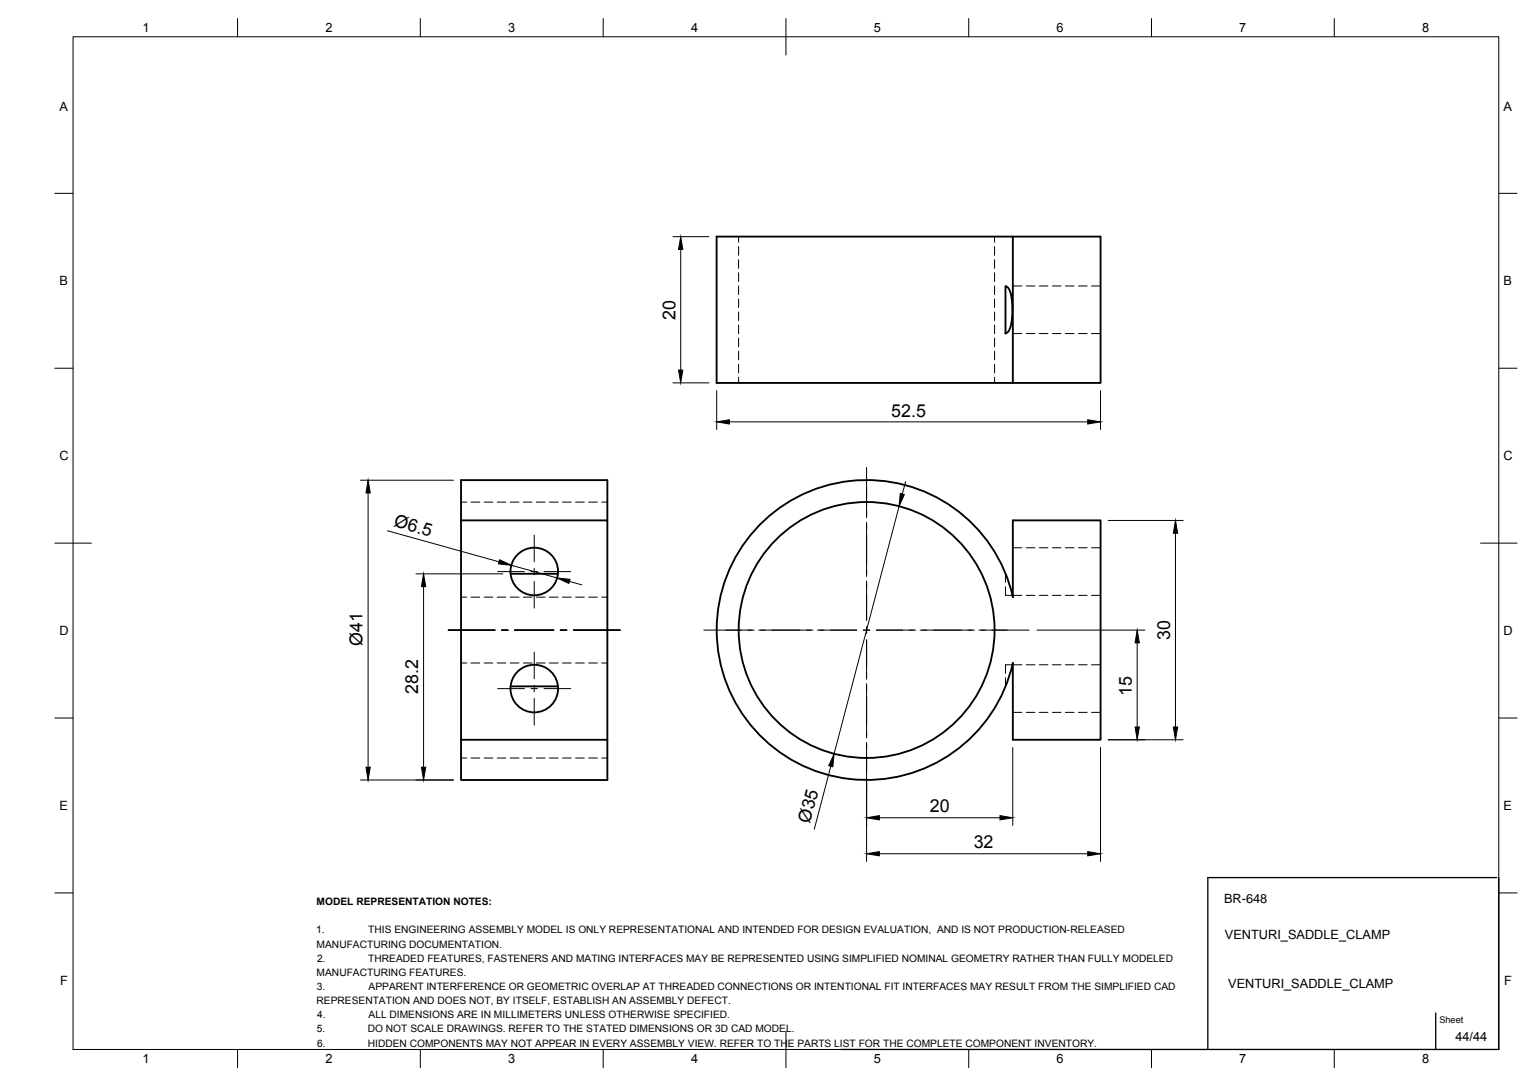
ISO-10303-21;
HEADER;
FILE_DESCRIPTION((''),'2;1');
FILE_NAME('VENTURI_SADDLE_CLAMP.step','2026-10-01T22:05:39-07:00',(''),(''),'','','');
FILE_SCHEMA (('AUTOMOTIVE_DESIGN { 1 0 10303 214 3 1 1 }'));
ENDSEC;
DATA;
#10=MECHANICAL_DESIGN_GEOMETRIC_PRESENTATION_REPRESENTATION('',(#640),#24628);
#556=SHAPE_REPRESENTATION_RELATIONSHIP('SRR','None',#24830,#598) ;
#598=ADVANCED_BREP_SHAPE_REPRESENTATION('',(#679),#24620) ;
#640=STYLED_ITEM('',(#25037),#679) ;
#679=MANIFOLD_SOLID_BREP('VENTURI_SADDLE_CLAMP',#13182) ;
#934=FACE_BOUND('',#4679,.T.) ;
#935=FACE_BOUND('',#4681,.T.) ;
#936=FACE_BOUND('',#4683,.T.) ;
#937=FACE_BOUND('',#4684,.T.) ;
#938=FACE_BOUND('',#4688,.T.) ;
#939=FACE_BOUND('',#4690,.T.) ;
#940=FACE_BOUND('',#4691,.T.) ;
#941=FACE_BOUND('',#4694,.T.) ;
#999=B_SPLINE_CURVE_WITH_KNOTS('',3,(#24196,#24197,#24198,#24199,#24200,
#24201,#24202,#24203,#24204,#24205,#24206,#24207,#24208,#24209,#24210,#24211,
#24212,#24213,#24214),.UNSPECIFIED.,.F.,.F.,(4,2,2,2,3,2,2,2,4),(-0.471793481292107,
-0.373843585675949,-0.243618913657373,-0.121809456828687,0.,0.121809456828687,
0.243618913657373,0.373843585675949,0.471793481292107),.UNSPECIFIED.) ;
#1000=B_SPLINE_CURVE_WITH_KNOTS('',3,(#24227,#24228,#24229,#24230,#24231,
#24232,#24233,#24234,#24235,#24236,#24237,#24238,#24239,#24240,#24241,#24242,
#24243,#24244),.UNSPECIFIED.,.F.,.F.,(4,2,2,2,2,2,2,2,4),(0.554019722357309,
0.651969617973467,0.782194289992043,0.904003746820729,1.02581320364942,
1.1476226604781,1.26943211730679,1.39965678932537,1.49760668494152),
 .UNSPECIFIED.) ;
#1736=LINE('',#24187,#2572) ;
#1737=LINE('',#24193,#2573) ;
#1738=LINE('',#24218,#2574) ;
#1739=LINE('',#24224,#2575) ;
#1740=LINE('',#24248,#2576) ;
#1741=LINE('',#24250,#2577) ;
#1742=LINE('',#24252,#2578) ;
#1743=LINE('',#24253,#2579) ;
#1744=LINE('',#24257,#2580) ;
#1745=LINE('',#24259,#2581) ;
#1746=LINE('',#24261,#2582) ;
#1747=LINE('',#24262,#2583) ;
#1748=LINE('',#24266,#2584) ;
#1749=LINE('',#24268,#2585) ;
#1750=LINE('',#24270,#2586) ;
#1751=LINE('',#24271,#2587) ;
#1752=LINE('',#24273,#2588) ;
#1753=LINE('',#24274,#2589) ;
#1754=LINE('',#24276,#2590) ;
#1755=LINE('',#24277,#2591) ;
#1756=LINE('',#24286,#2592) ;
#2572=VECTOR('',#19353,1.) ;
#2573=VECTOR('',#19360,0.325) ;
#2574=VECTOR('',#19367,1.) ;
#2575=VECTOR('',#19374,0.325) ;
#2576=VECTOR('',#19381,1.) ;
#2577=VECTOR('',#19382,1.) ;
#2578=VECTOR('',#19383,1.) ;
#2579=VECTOR('',#19384,1.) ;
#2580=VECTOR('',#19387,1.) ;
#2581=VECTOR('',#19388,1.) ;
#2582=VECTOR('',#19389,1.) ;
#2583=VECTOR('',#19390,1.) ;
#2584=VECTOR('',#19393,1.) ;
#2585=VECTOR('',#19394,1.) ;
#2586=VECTOR('',#19395,1.) ;
#2587=VECTOR('',#19396,1.) ;
#2588=VECTOR('',#19399,1.) ;
#2589=VECTOR('',#19400,1.) ;
#2590=VECTOR('',#19403,1.) ;
#2591=VECTOR('',#19404,1.) ;
#2592=VECTOR('',#19417,1.75) ;
#2938=CYLINDRICAL_SURFACE('',#15267,0.325) ;
#2939=CYLINDRICAL_SURFACE('',#15270,0.325) ;
#2940=CYLINDRICAL_SURFACE('',#15273,0.325) ;
#2941=CYLINDRICAL_SURFACE('',#15276,0.325) ;
#2942=CYLINDRICAL_SURFACE('',#15285,2.05) ;
#2943=CYLINDRICAL_SURFACE('',#15287,1.75) ;
#3657=FACE_OUTER_BOUND('',#4672,.T.) ;
#3658=FACE_OUTER_BOUND('',#4673,.T.) ;
#3659=FACE_OUTER_BOUND('',#4674,.T.) ;
#3660=FACE_OUTER_BOUND('',#4675,.T.) ;
#3661=FACE_OUTER_BOUND('',#4676,.T.) ;
#3662=FACE_OUTER_BOUND('',#4677,.T.) ;
#3663=FACE_OUTER_BOUND('',#4678,.T.) ;
#3664=FACE_OUTER_BOUND('',#4680,.T.) ;
#3665=FACE_OUTER_BOUND('',#4682,.T.) ;
#3666=FACE_OUTER_BOUND('',#4685,.T.) ;
#3667=FACE_OUTER_BOUND('',#4686,.T.) ;
#3668=FACE_OUTER_BOUND('',#4687,.T.) ;
#3669=FACE_OUTER_BOUND('',#4689,.T.) ;
#3670=FACE_OUTER_BOUND('',#4692,.T.) ;
#3671=FACE_OUTER_BOUND('',#4693,.T.) ;
#4672=EDGE_LOOP('',(#11737,#11738)) ;
#4673=EDGE_LOOP('',(#11739,#11740,#11741,#11742)) ;
#4674=EDGE_LOOP('',(#11743,#11744)) ;
#4675=EDGE_LOOP('',(#11745,#11746)) ;
#4676=EDGE_LOOP('',(#11747,#11748,#11749,#11750)) ;
#4677=EDGE_LOOP('',(#11751,#11752)) ;
#4678=EDGE_LOOP('',(#11753,#11754,#11755,#11756)) ;
#4679=EDGE_LOOP('',(#11757)) ;
#4680=EDGE_LOOP('',(#11758,#11759,#11760,#11761)) ;
#4681=EDGE_LOOP('',(#11762)) ;
#4682=EDGE_LOOP('',(#11763,#11764,#11765,#11766)) ;
#4683=EDGE_LOOP('',(#11767)) ;
#4684=EDGE_LOOP('',(#11768)) ;
#4685=EDGE_LOOP('',(#11769,#11770,#11771,#11772)) ;
#4686=EDGE_LOOP('',(#11773,#11774,#11775,#11776)) ;
#4687=EDGE_LOOP('',(#11777,#11778,#11779,#11780,#11781,#11782)) ;
#4688=EDGE_LOOP('',(#11783)) ;
#4689=EDGE_LOOP('',(#11784,#11785,#11786,#11787)) ;
#4690=EDGE_LOOP('',(#11788,#11789)) ;
#4691=EDGE_LOOP('',(#11790,#11791)) ;
#4692=EDGE_LOOP('',(#11792,#11793,#11794,#11795)) ;
#4693=EDGE_LOOP('',(#11796,#11797,#11798,#11799,#11800,#11801)) ;
#4694=EDGE_LOOP('',(#11802)) ;
#5511=CIRCLE('',#15266,0.325) ;
#5512=CIRCLE('',#15268,0.325) ;
#5513=CIRCLE('',#15269,0.325) ;
#5514=CIRCLE('',#15272,0.325) ;
#5515=CIRCLE('',#15274,0.325) ;
#5516=CIRCLE('',#15275,0.325) ;
#5517=CIRCLE('',#15283,2.05) ;
#5518=CIRCLE('',#15284,1.75) ;
#5519=CIRCLE('',#15286,2.05) ;
#5520=CIRCLE('',#15288,1.75) ;
#6647=VERTEX_POINT('',#24185) ;
#6648=VERTEX_POINT('',#24186) ;
#6649=VERTEX_POINT('',#24190) ;
#6650=VERTEX_POINT('',#24192) ;
#6651=VERTEX_POINT('',#24216) ;
#6652=VERTEX_POINT('',#24217) ;
#6653=VERTEX_POINT('',#24221) ;
#6654=VERTEX_POINT('',#24223) ;
#6655=VERTEX_POINT('',#24246) ;
#6656=VERTEX_POINT('',#24247) ;
#6657=VERTEX_POINT('',#24249) ;
#6658=VERTEX_POINT('',#24251) ;
#6659=VERTEX_POINT('',#24255) ;
#6660=VERTEX_POINT('',#24256) ;
#6661=VERTEX_POINT('',#24258) ;
#6662=VERTEX_POINT('',#24260) ;
#6663=VERTEX_POINT('',#24264) ;
#6664=VERTEX_POINT('',#24265) ;
#6665=VERTEX_POINT('',#24267) ;
#6666=VERTEX_POINT('',#24269) ;
#6667=VERTEX_POINT('',#24280) ;
#6668=VERTEX_POINT('',#24285) ;
#8358=EDGE_CURVE('',#6647,#6648,#1736,.T.) ;
#8359=EDGE_CURVE('',#6648,#6647,#5511,.T.) ;
#8360=EDGE_CURVE('',#6649,#6649,#5512,.T.) ;
#8361=EDGE_CURVE('',#6649,#6650,#1737,.T.) ;
#8362=EDGE_CURVE('',#6650,#6650,#5513,.T.) ;
#8363=EDGE_CURVE('',#6648,#6647,#999,.T.) ;
#8364=EDGE_CURVE('',#6651,#6652,#1738,.T.) ;
#8365=EDGE_CURVE('',#6652,#6651,#5514,.T.) ;
#8366=EDGE_CURVE('',#6653,#6653,#5515,.T.) ;
#8367=EDGE_CURVE('',#6653,#6654,#1739,.T.) ;
#8368=EDGE_CURVE('',#6654,#6654,#5516,.T.) ;
#8369=EDGE_CURVE('',#6652,#6651,#1000,.T.) ;
#8370=EDGE_CURVE('',#6655,#6656,#1740,.T.) ;
#8371=EDGE_CURVE('',#6655,#6657,#1741,.T.) ;
#8372=EDGE_CURVE('',#6657,#6658,#1742,.T.) ;
#8373=EDGE_CURVE('',#6658,#6656,#1743,.T.) ;
#8374=EDGE_CURVE('',#6659,#6660,#1744,.T.) ;
#8375=EDGE_CURVE('',#6659,#6661,#1745,.T.) ;
#8376=EDGE_CURVE('',#6661,#6662,#1746,.T.) ;
#8377=EDGE_CURVE('',#6662,#6660,#1747,.T.) ;
#8378=EDGE_CURVE('',#6663,#6664,#1748,.T.) ;
#8379=EDGE_CURVE('',#6664,#6665,#1749,.T.) ;
#8380=EDGE_CURVE('',#6665,#6666,#1750,.T.) ;
#8381=EDGE_CURVE('',#6666,#6663,#1751,.T.) ;
#8382=EDGE_CURVE('',#6657,#6665,#1752,.T.) ;
#8383=EDGE_CURVE('',#6658,#6664,#1753,.T.) ;
#8384=EDGE_CURVE('',#6661,#6663,#1754,.T.) ;
#8385=EDGE_CURVE('',#6662,#6666,#1755,.T.) ;
#8386=EDGE_CURVE('',#6655,#6660,#5517,.T.) ;
#8387=EDGE_CURVE('',#6667,#6667,#5518,.T.) ;
#8388=EDGE_CURVE('',#6659,#6656,#5519,.T.) ;
#8389=EDGE_CURVE('',#6667,#6668,#1756,.T.) ;
#8390=EDGE_CURVE('',#6668,#6668,#5520,.T.) ;
#11737=ORIENTED_EDGE('',*,*,#8358,.F.) ;
#11738=ORIENTED_EDGE('',*,*,#8359,.F.) ;
#11739=ORIENTED_EDGE('',*,*,#8360,.F.) ;
#11740=ORIENTED_EDGE('',*,*,#8361,.T.) ;
#11741=ORIENTED_EDGE('',*,*,#8362,.F.) ;
#11742=ORIENTED_EDGE('',*,*,#8361,.F.) ;
#11743=ORIENTED_EDGE('',*,*,#8363,.F.) ;
#11744=ORIENTED_EDGE('',*,*,#8359,.T.) ;
#11745=ORIENTED_EDGE('',*,*,#8364,.F.) ;
#11746=ORIENTED_EDGE('',*,*,#8365,.F.) ;
#11747=ORIENTED_EDGE('',*,*,#8366,.F.) ;
#11748=ORIENTED_EDGE('',*,*,#8367,.T.) ;
#11749=ORIENTED_EDGE('',*,*,#8368,.F.) ;
#11750=ORIENTED_EDGE('',*,*,#8367,.F.) ;
#11751=ORIENTED_EDGE('',*,*,#8369,.F.) ;
#11752=ORIENTED_EDGE('',*,*,#8365,.T.) ;
#11753=ORIENTED_EDGE('',*,*,#8370,.F.) ;
#11754=ORIENTED_EDGE('',*,*,#8371,.T.) ;
#11755=ORIENTED_EDGE('',*,*,#8372,.T.) ;
#11756=ORIENTED_EDGE('',*,*,#8373,.T.) ;
#11757=ORIENTED_EDGE('',*,*,#8368,.T.) ;
#11758=ORIENTED_EDGE('',*,*,#8374,.F.) ;
#11759=ORIENTED_EDGE('',*,*,#8375,.T.) ;
#11760=ORIENTED_EDGE('',*,*,#8376,.T.) ;
#11761=ORIENTED_EDGE('',*,*,#8377,.T.) ;
#11762=ORIENTED_EDGE('',*,*,#8362,.T.) ;
#11763=ORIENTED_EDGE('',*,*,#8378,.T.) ;
#11764=ORIENTED_EDGE('',*,*,#8379,.T.) ;
#11765=ORIENTED_EDGE('',*,*,#8380,.T.) ;
#11766=ORIENTED_EDGE('',*,*,#8381,.T.) ;
#11767=ORIENTED_EDGE('',*,*,#8360,.T.) ;
#11768=ORIENTED_EDGE('',*,*,#8366,.T.) ;
#11769=ORIENTED_EDGE('',*,*,#8382,.T.) ;
#11770=ORIENTED_EDGE('',*,*,#8379,.F.) ;
#11771=ORIENTED_EDGE('',*,*,#8383,.F.) ;
#11772=ORIENTED_EDGE('',*,*,#8372,.F.) ;
#11773=ORIENTED_EDGE('',*,*,#8384,.T.) ;
#11774=ORIENTED_EDGE('',*,*,#8381,.F.) ;
#11775=ORIENTED_EDGE('',*,*,#8385,.F.) ;
#11776=ORIENTED_EDGE('',*,*,#8376,.F.) ;
#11777=ORIENTED_EDGE('',*,*,#8386,.T.) ;
#11778=ORIENTED_EDGE('',*,*,#8377,.F.) ;
#11779=ORIENTED_EDGE('',*,*,#8385,.T.) ;
#11780=ORIENTED_EDGE('',*,*,#8380,.F.) ;
#11781=ORIENTED_EDGE('',*,*,#8382,.F.) ;
#11782=ORIENTED_EDGE('',*,*,#8371,.F.) ;
#11783=ORIENTED_EDGE('',*,*,#8387,.T.) ;
#11784=ORIENTED_EDGE('',*,*,#8374,.T.) ;
#11785=ORIENTED_EDGE('',*,*,#8386,.F.) ;
#11786=ORIENTED_EDGE('',*,*,#8370,.T.) ;
#11787=ORIENTED_EDGE('',*,*,#8388,.F.) ;
#11788=ORIENTED_EDGE('',*,*,#8363,.T.) ;
#11789=ORIENTED_EDGE('',*,*,#8358,.T.) ;
#11790=ORIENTED_EDGE('',*,*,#8369,.T.) ;
#11791=ORIENTED_EDGE('',*,*,#8364,.T.) ;
#11792=ORIENTED_EDGE('',*,*,#8387,.F.) ;
#11793=ORIENTED_EDGE('',*,*,#8389,.T.) ;
#11794=ORIENTED_EDGE('',*,*,#8390,.F.) ;
#11795=ORIENTED_EDGE('',*,*,#8389,.F.) ;
#11796=ORIENTED_EDGE('',*,*,#8388,.T.) ;
#11797=ORIENTED_EDGE('',*,*,#8373,.F.) ;
#11798=ORIENTED_EDGE('',*,*,#8383,.T.) ;
#11799=ORIENTED_EDGE('',*,*,#8378,.F.) ;
#11800=ORIENTED_EDGE('',*,*,#8384,.F.) ;
#11801=ORIENTED_EDGE('',*,*,#8375,.F.) ;
#11802=ORIENTED_EDGE('',*,*,#8390,.T.) ;
#12299=PLANE('',#15265) ;
#12300=PLANE('',#15271) ;
#12301=PLANE('',#15277) ;
#12302=PLANE('',#15278) ;
#12303=PLANE('',#15279) ;
#12304=PLANE('',#15280) ;
#12305=PLANE('',#15281) ;
#12306=PLANE('',#15282) ;
#12307=PLANE('',#15289) ;
#13052=ADVANCED_FACE('',(#3657),#12299,.F.) ;
#13053=ADVANCED_FACE('',(#3658),#2938,.F.) ;
#13054=ADVANCED_FACE('',(#3659),#2939,.F.) ;
#13055=ADVANCED_FACE('',(#3660),#12300,.F.) ;
#13056=ADVANCED_FACE('',(#3661),#2940,.F.) ;
#13057=ADVANCED_FACE('',(#3662),#2941,.F.) ;
#13058=ADVANCED_FACE('',(#3663,#934),#12301,.T.) ;
#13059=ADVANCED_FACE('',(#3664,#935),#12302,.T.) ;
#13060=ADVANCED_FACE('',(#3665,#936,#937),#12303,.F.) ;
#13061=ADVANCED_FACE('',(#3666),#12304,.F.) ;
#13062=ADVANCED_FACE('',(#3667),#12305,.F.) ;
#13063=ADVANCED_FACE('',(#3668,#938),#12306,.T.) ;
#13064=ADVANCED_FACE('',(#3669,#939,#940),#2942,.T.) ;
#13065=ADVANCED_FACE('',(#3670),#2943,.F.) ;
#13066=ADVANCED_FACE('',(#3671,#941),#12307,.T.) ;
#13182=CLOSED_SHELL('',(#13052,#13053,#13054,#13055,#13056,#13057,#13058,
#13059,#13060,#13061,#13062,#13063,#13064,#13065,#13066)) ;
#15264=AXIS2_PLACEMENT_3D('',#24183,#19349,#19350) ;
#15265=AXIS2_PLACEMENT_3D('',#24184,#19351,#19352) ;
#15266=AXIS2_PLACEMENT_3D('',#24188,#19354,#19355) ;
#15267=AXIS2_PLACEMENT_3D('',#24189,#19356,#19357) ;
#15268=AXIS2_PLACEMENT_3D('',#24191,#19358,#19359) ;
#15269=AXIS2_PLACEMENT_3D('',#24194,#19361,#19362) ;
#15270=AXIS2_PLACEMENT_3D('',#24195,#19363,#19364) ;
#15271=AXIS2_PLACEMENT_3D('',#24215,#19365,#19366) ;
#15272=AXIS2_PLACEMENT_3D('',#24219,#19368,#19369) ;
#15273=AXIS2_PLACEMENT_3D('',#24220,#19370,#19371) ;
#15274=AXIS2_PLACEMENT_3D('',#24222,#19372,#19373) ;
#15275=AXIS2_PLACEMENT_3D('',#24225,#19375,#19376) ;
#15276=AXIS2_PLACEMENT_3D('',#24226,#19377,#19378) ;
#15277=AXIS2_PLACEMENT_3D('',#24245,#19379,#19380) ;
#15278=AXIS2_PLACEMENT_3D('',#24254,#19385,#19386) ;
#15279=AXIS2_PLACEMENT_3D('',#24263,#19391,#19392) ;
#15280=AXIS2_PLACEMENT_3D('',#24272,#19397,#19398) ;
#15281=AXIS2_PLACEMENT_3D('',#24275,#19401,#19402) ;
#15282=AXIS2_PLACEMENT_3D('',#24278,#19405,#19406) ;
#15283=AXIS2_PLACEMENT_3D('',#24279,#19407,#19408) ;
#15284=AXIS2_PLACEMENT_3D('',#24281,#19409,#19410) ;
#15285=AXIS2_PLACEMENT_3D('',#24282,#19411,#19412) ;
#15286=AXIS2_PLACEMENT_3D('',#24283,#19413,#19414) ;
#15287=AXIS2_PLACEMENT_3D('',#24284,#19415,#19416) ;
#15288=AXIS2_PLACEMENT_3D('',#24287,#19418,#19419) ;
#15289=AXIS2_PLACEMENT_3D('',#24288,#19420,#19421) ;
#19349=DIRECTION('axis',(0.,0.,1.)) ;
#19350=DIRECTION('refdir',(1.,0.,0.)) ;
#19351=DIRECTION('center_axis',(0.,0.,1.)) ;
#19352=DIRECTION('ref_axis',(1.,0.,0.)) ;
#19353=DIRECTION('',(-1.,0.,0.)) ;
#19354=DIRECTION('center_axis',(0.,0.,1.)) ;
#19355=DIRECTION('ref_axis',(1.,0.,0.)) ;
#19356=DIRECTION('center_axis',(0.,0.,1.)) ;
#19357=DIRECTION('ref_axis',(1.,0.,0.)) ;
#19358=DIRECTION('center_axis',(0.,0.,1.)) ;
#19359=DIRECTION('ref_axis',(1.,0.,0.)) ;
#19360=DIRECTION('',(0.,0.,1.)) ;
#19361=DIRECTION('center_axis',(0.,0.,-1.)) ;
#19362=DIRECTION('ref_axis',(1.,0.,0.)) ;
#19363=DIRECTION('center_axis',(0.,0.,1.)) ;
#19364=DIRECTION('ref_axis',(1.,0.,0.)) ;
#19365=DIRECTION('center_axis',(0.,0.,1.)) ;
#19366=DIRECTION('ref_axis',(1.,0.,0.)) ;
#19367=DIRECTION('',(1.,0.,0.)) ;
#19368=DIRECTION('center_axis',(0.,0.,1.)) ;
#19369=DIRECTION('ref_axis',(1.,0.,0.)) ;
#19370=DIRECTION('center_axis',(0.,0.,1.)) ;
#19371=DIRECTION('ref_axis',(1.,0.,0.)) ;
#19372=DIRECTION('center_axis',(0.,0.,1.)) ;
#19373=DIRECTION('ref_axis',(1.,0.,0.)) ;
#19374=DIRECTION('',(0.,0.,1.)) ;
#19375=DIRECTION('center_axis',(0.,0.,-1.)) ;
#19376=DIRECTION('ref_axis',(1.,0.,0.)) ;
#19377=DIRECTION('center_axis',(0.,0.,1.)) ;
#19378=DIRECTION('ref_axis',(1.,0.,0.)) ;
#19379=DIRECTION('center_axis',(0.,0.,1.)) ;
#19380=DIRECTION('ref_axis',(1.,0.,0.)) ;
#19381=DIRECTION('',(1.,0.,0.)) ;
#19382=DIRECTION('',(0.,-1.,0.)) ;
#19383=DIRECTION('',(1.,0.,0.)) ;
#19384=DIRECTION('',(0.,1.,0.)) ;
#19385=DIRECTION('center_axis',(0.,0.,1.)) ;
#19386=DIRECTION('ref_axis',(1.,0.,0.)) ;
#19387=DIRECTION('',(-1.,0.,0.)) ;
#19388=DIRECTION('',(0.,1.,0.)) ;
#19389=DIRECTION('',(-1.,0.,0.)) ;
#19390=DIRECTION('',(0.,-1.,0.)) ;
#19391=DIRECTION('center_axis',(0.,0.,1.)) ;
#19392=DIRECTION('ref_axis',(1.,0.,0.)) ;
#19393=DIRECTION('',(0.,-1.,0.)) ;
#19394=DIRECTION('',(-1.,0.,0.)) ;
#19395=DIRECTION('',(0.,1.,0.)) ;
#19396=DIRECTION('',(1.,0.,0.)) ;
#19397=DIRECTION('center_axis',(0.,1.,0.)) ;
#19398=DIRECTION('ref_axis',(0.,0.,1.)) ;
#19399=DIRECTION('',(0.,0.,-1.)) ;
#19400=DIRECTION('',(0.,0.,-1.)) ;
#19401=DIRECTION('center_axis',(0.,-1.,0.)) ;
#19402=DIRECTION('ref_axis',(0.,0.,-1.)) ;
#19403=DIRECTION('',(0.,0.,-1.)) ;
#19404=DIRECTION('',(0.,0.,-1.)) ;
#19405=DIRECTION('center_axis',(-1.,0.,0.)) ;
#19406=DIRECTION('ref_axis',(0.,0.,1.)) ;
#19407=DIRECTION('center_axis',(-1.,0.,0.)) ;
#19408=DIRECTION('ref_axis',(0.,0.,-1.)) ;
#19409=DIRECTION('center_axis',(1.,0.,0.)) ;
#19410=DIRECTION('ref_axis',(0.,0.,-1.)) ;
#19411=DIRECTION('center_axis',(1.,0.,0.)) ;
#19412=DIRECTION('ref_axis',(0.,1.22464679914735E-16,1.)) ;
#19413=DIRECTION('center_axis',(1.,0.,0.)) ;
#19414=DIRECTION('ref_axis',(0.,0.,-1.)) ;
#19415=DIRECTION('center_axis',(1.,0.,0.)) ;
#19416=DIRECTION('ref_axis',(0.,0.,-1.)) ;
#19417=DIRECTION('',(1.,0.,0.)) ;
#19418=DIRECTION('center_axis',(-1.,0.,0.)) ;
#19419=DIRECTION('ref_axis',(0.,0.,-1.)) ;
#19420=DIRECTION('center_axis',(1.,0.,0.)) ;
#19421=DIRECTION('ref_axis',(0.,0.,-1.)) ;
#24183=CARTESIAN_POINT('',(0.,0.,0.)) ;
#24184=CARTESIAN_POINT('Origin',(0.,-1.,-18.4)) ;
#24185=CARTESIAN_POINT('',(0.32358823443885,-1.03025978408297,-18.4)) ;
#24186=CARTESIAN_POINT('',(-0.32358823443885,-1.03025978408297,-18.4)) ;
#24187=CARTESIAN_POINT('',(0.,-1.03025978408297,-18.4)) ;
#24188=CARTESIAN_POINT('Origin',(0.,-1.,-18.4)) ;
#24189=CARTESIAN_POINT('Origin',(0.,-1.,-19.1)) ;
#24190=CARTESIAN_POINT('',(-0.325,-1.,-19.7)) ;
#24191=CARTESIAN_POINT('Origin',(0.,-1.,-19.7)) ;
#24192=CARTESIAN_POINT('',(-0.325,-1.,-18.5)) ;
#24193=CARTESIAN_POINT('',(-0.325,-1.,-19.1)) ;
#24194=CARTESIAN_POINT('Origin',(0.,-1.,-18.5)) ;
#24195=CARTESIAN_POINT('Origin',(0.,-1.,-19.1)) ;
#24196=CARTESIAN_POINT('Ctrl Pts',(-0.32358823443885,-1.03025978408297,
-18.4)) ;
#24197=CARTESIAN_POINT('Ctrl Pts',(-0.320683284716929,-1.06132436633751,
-18.4125850832905)) ;
#24198=CARTESIAN_POINT('Ctrl Pts',(-0.313012256587164,-1.093473322376,-18.4246724562692)) ;
#24199=CARTESIAN_POINT('Ctrl Pts',(-0.283688317673296,-1.16453182056614,
-18.4494936673328)) ;
#24200=CARTESIAN_POINT('Ctrl Pts',(-0.258016677129131,-1.20214547201537,
-18.4611303131333)) ;
#24201=CARTESIAN_POINT('Ctrl Pts',(-0.199245732245778,-1.25982709091893,
-18.4777651627884)) ;
#24202=CARTESIAN_POINT('Ctrl Pts',(-0.16316880358915,-1.28432292672745,
-18.4841520686026)) ;
#24203=CARTESIAN_POINT('Ctrl Pts',(-0.0838450021535121,-1.31691261760816,
-18.4923375343137)) ;
#24204=CARTESIAN_POINT('Ctrl Pts',(-0.0406031522762289,-1.325,-18.4942103700463)) ;
#24205=CARTESIAN_POINT('Ctrl Pts',(0.,-1.325,-18.4942103700463)) ;
#24206=CARTESIAN_POINT('Ctrl Pts',(0.0406031522762288,-1.325,-18.4942103700463)) ;
#24207=CARTESIAN_POINT('Ctrl Pts',(0.083845002153512,-1.31691261760816,
-18.4923375343137)) ;
#24208=CARTESIAN_POINT('Ctrl Pts',(0.16316880358915,-1.28432292672745,-18.4841520686026)) ;
#24209=CARTESIAN_POINT('Ctrl Pts',(0.199245732245778,-1.25982709091893,
-18.4777651627884)) ;
#24210=CARTESIAN_POINT('Ctrl Pts',(0.258016677129131,-1.20214547201537,
-18.4611303131333)) ;
#24211=CARTESIAN_POINT('Ctrl Pts',(0.283688317673296,-1.16453182056614,
-18.4494936673328)) ;
#24212=CARTESIAN_POINT('Ctrl Pts',(0.313012256587164,-1.093473322376,-18.4246724562692)) ;
#24213=CARTESIAN_POINT('Ctrl Pts',(0.320683284716929,-1.06132436633751,
-18.4125850832905)) ;
#24214=CARTESIAN_POINT('Ctrl Pts',(0.32358823443885,-1.03025978408297,-18.4)) ;
#24215=CARTESIAN_POINT('Origin',(0.,-2.6,-18.4)) ;
#24216=CARTESIAN_POINT('',(-0.32358823443885,-2.56974021591703,-18.4)) ;
#24217=CARTESIAN_POINT('',(0.32358823443885,-2.56974021591703,-18.4)) ;
#24218=CARTESIAN_POINT('',(0.,-2.56974021591703,-18.4)) ;
#24219=CARTESIAN_POINT('Origin',(0.,-2.6,-18.4)) ;
#24220=CARTESIAN_POINT('Origin',(0.,-2.6,-19.1)) ;
#24221=CARTESIAN_POINT('',(-0.325,-2.6,-19.7)) ;
#24222=CARTESIAN_POINT('Origin',(0.,-2.6,-19.7)) ;
#24223=CARTESIAN_POINT('',(-0.325,-2.6,-18.5)) ;
#24224=CARTESIAN_POINT('',(-0.325,-2.6,-19.1)) ;
#24225=CARTESIAN_POINT('Origin',(0.,-2.6,-18.5)) ;
#24226=CARTESIAN_POINT('Origin',(0.,-2.6,-19.1)) ;
#24227=CARTESIAN_POINT('Ctrl Pts',(0.32358823443885,-2.56974021591703,-18.4)) ;
#24228=CARTESIAN_POINT('Ctrl Pts',(0.320683284716929,-2.53867563366249,
-18.4125850832905)) ;
#24229=CARTESIAN_POINT('Ctrl Pts',(0.313012256587164,-2.506526677624,-18.4246724562692)) ;
#24230=CARTESIAN_POINT('Ctrl Pts',(0.283688317673296,-2.43546817943386,
-18.4494936673328)) ;
#24231=CARTESIAN_POINT('Ctrl Pts',(0.258016677129131,-2.39785452798463,
-18.4611303131333)) ;
#24232=CARTESIAN_POINT('Ctrl Pts',(0.199245732245778,-2.34017290908107,
-18.4777651627884)) ;
#24233=CARTESIAN_POINT('Ctrl Pts',(0.16316880358915,-2.31567707327255,-18.4841520686026)) ;
#24234=CARTESIAN_POINT('Ctrl Pts',(0.0838450021535119,-2.28308738239184,
-18.4923375343137)) ;
#24235=CARTESIAN_POINT('Ctrl Pts',(0.0406031522762289,-2.275,-18.4942103700463)) ;
#24236=CARTESIAN_POINT('Ctrl Pts',(-0.0406031522762288,-2.275,-18.4942103700463)) ;
#24237=CARTESIAN_POINT('Ctrl Pts',(-0.0838450021535119,-2.28308738239184,
-18.4923375343137)) ;
#24238=CARTESIAN_POINT('Ctrl Pts',(-0.16316880358915,-2.31567707327255,
-18.4841520686026)) ;
#24239=CARTESIAN_POINT('Ctrl Pts',(-0.199245732245778,-2.34017290908107,
-18.4777651627884)) ;
#24240=CARTESIAN_POINT('Ctrl Pts',(-0.258016677129131,-2.39785452798463,
-18.4611303131333)) ;
#24241=CARTESIAN_POINT('Ctrl Pts',(-0.283688317673296,-2.43546817943386,
-18.4494936673328)) ;
#24242=CARTESIAN_POINT('Ctrl Pts',(-0.313012256587164,-2.506526677624,-18.4246724562692)) ;
#24243=CARTESIAN_POINT('Ctrl Pts',(-0.320683284716929,-2.53867563366249,
-18.4125850832905)) ;
#24244=CARTESIAN_POINT('Ctrl Pts',(-0.32358823443885,-2.56974021591703,
-18.4)) ;
#24245=CARTESIAN_POINT('Origin',(0.,-1.8,-18.5)) ;
#24246=CARTESIAN_POINT('',(-1.,-2.25,-18.5)) ;
#24247=CARTESIAN_POINT('',(1.,-2.25,-18.5)) ;
#24248=CARTESIAN_POINT('',(0.,-2.25,-18.5)) ;
#24249=CARTESIAN_POINT('',(-1.,-3.3,-18.5)) ;
#24250=CARTESIAN_POINT('',(-1.,-1.8,-18.5)) ;
#24251=CARTESIAN_POINT('',(1.,-3.3,-18.5)) ;
#24252=CARTESIAN_POINT('',(0.,-3.3,-18.5)) ;
#24253=CARTESIAN_POINT('',(1.,-1.8,-18.5)) ;
#24254=CARTESIAN_POINT('Origin',(0.,-1.8,-18.5)) ;
#24255=CARTESIAN_POINT('',(1.,-1.35,-18.5)) ;
#24256=CARTESIAN_POINT('',(-1.,-1.35,-18.5)) ;
#24257=CARTESIAN_POINT('',(0.,-1.35,-18.5)) ;
#24258=CARTESIAN_POINT('',(1.,-0.3,-18.5)) ;
#24259=CARTESIAN_POINT('',(1.,-1.8,-18.5)) ;
#24260=CARTESIAN_POINT('',(-1.,-0.3,-18.5)) ;
#24261=CARTESIAN_POINT('',(0.,-0.3,-18.5)) ;
#24262=CARTESIAN_POINT('',(-1.,-1.8,-18.5)) ;
#24263=CARTESIAN_POINT('Origin',(0.,-1.8,-19.7)) ;
#24264=CARTESIAN_POINT('',(1.,-0.3,-19.7)) ;
#24265=CARTESIAN_POINT('',(1.,-3.3,-19.7)) ;
#24266=CARTESIAN_POINT('',(1.,-1.8,-19.7)) ;
#24267=CARTESIAN_POINT('',(-1.,-3.3,-19.7)) ;
#24268=CARTESIAN_POINT('',(0.,-3.3,-19.7)) ;
#24269=CARTESIAN_POINT('',(-1.,-0.3,-19.7)) ;
#24270=CARTESIAN_POINT('',(-1.,-1.8,-19.7)) ;
#24271=CARTESIAN_POINT('',(0.,-0.3,-19.7)) ;
#24272=CARTESIAN_POINT('Origin',(0.,-3.3,-19.1)) ;
#24273=CARTESIAN_POINT('',(-1.,-3.3,-19.1)) ;
#24274=CARTESIAN_POINT('',(1.,-3.3,-19.1)) ;
#24275=CARTESIAN_POINT('Origin',(0.,-0.3,-19.1)) ;
#24276=CARTESIAN_POINT('',(1.,-0.3,-19.1)) ;
#24277=CARTESIAN_POINT('',(-1.,-0.3,-19.1)) ;
#24278=CARTESIAN_POINT('Origin',(-1.,-1.8,-16.5)) ;
#24279=CARTESIAN_POINT('Origin',(-1.,-1.8,-16.5)) ;
#24280=CARTESIAN_POINT('',(-1.,-1.8,-14.75)) ;
#24281=CARTESIAN_POINT('Origin',(-1.,-1.8,-16.5)) ;
#24282=CARTESIAN_POINT('Origin',(0.,-1.8,-16.5)) ;
#24283=CARTESIAN_POINT('Origin',(1.,-1.8,-16.5)) ;
#24284=CARTESIAN_POINT('Origin',(0.,-1.8,-16.5)) ;
#24285=CARTESIAN_POINT('',(1.,-1.8,-14.75)) ;
#24286=CARTESIAN_POINT('',(0.,-1.8,-14.75)) ;
#24287=CARTESIAN_POINT('Origin',(1.,-1.8,-16.5)) ;
#24288=CARTESIAN_POINT('Origin',(1.,-1.8,-16.5)) ;
#24572=UNCERTAINTY_MEASURE_WITH_UNIT(LENGTH_MEASURE(0.001),#24629,
'DISTANCE_ACCURACY_VALUE',
'Maximum model space distance between geometric entities at asserted c
onnectivities') ;
#24580=UNCERTAINTY_MEASURE_WITH_UNIT(LENGTH_MEASURE(0.001),#24629,
'DISTANCE_ACCURACY_VALUE',
'Maximum model space distance between geometric entities at asserted c
onnectivities') ;
#24620=(
GEOMETRIC_REPRESENTATION_CONTEXT(3)
GLOBAL_UNCERTAINTY_ASSIGNED_CONTEXT((#24572))
GLOBAL_UNIT_ASSIGNED_CONTEXT((#24629,#24631,#24632))
REPRESENTATION_CONTEXT('','3D')
) ;
#24628=(
GEOMETRIC_REPRESENTATION_CONTEXT(3)
GLOBAL_UNCERTAINTY_ASSIGNED_CONTEXT((#24580))
GLOBAL_UNIT_ASSIGNED_CONTEXT((#24629,#24631,#24632))
REPRESENTATION_CONTEXT('','3D')
) ;
#24629=(
LENGTH_UNIT()
NAMED_UNIT(*)
SI_UNIT(.CENTI.,.METRE.)
) ;
#24631=(
NAMED_UNIT(*)
PLANE_ANGLE_UNIT()
SI_UNIT($,.RADIAN.)
) ;
#24632=(
NAMED_UNIT(*)
SI_UNIT($,.STERADIAN.)
SOLID_ANGLE_UNIT()
) ;
#24672=SHAPE_DEFINITION_REPRESENTATION(#24753,#24830) ;
#24753=PRODUCT_DEFINITION_SHAPE('',$,#24878) ;
#24830=SHAPE_REPRESENTATION('',(#15264),#24620) ;
#24838=PRODUCT_DEFINITION_CONTEXT('part definition',#24981,'design') ;
#24878=PRODUCT_DEFINITION('VENTURI_SADDLE_CLAMP',
'VENTURI_SADDLE_CLAMP',#24925,#24838) ;
#24925=PRODUCT_DEFINITION_FORMATION('',$,#25022) ;
#24981=APPLICATION_CONTEXT(
'Core Data for Automotive Mechanical Design Process') ;
#24982=PRODUCT_CONTEXT('part definition',#24981,'mechanical') ;
#25022=PRODUCT('VENTURI_SADDLE_CLAMP','VENTURI_SADDLE_CLAMP',$,(#24982)) ;
#25037=PRESENTATION_STYLE_ASSIGNMENT((#25047)) ;
#25047=SURFACE_STYLE_USAGE(.BOTH.,#25057) ;
#25057=SURFACE_SIDE_STYLE('',(#25067)) ;
#25067=SURFACE_STYLE_FILL_AREA(#25077) ;
#25077=FILL_AREA_STYLE('Steel - Galvanized (Small)',(#25087)) ;
#25087=FILL_AREA_STYLE_COLOUR('Steel - Galvanized (Small)',#25097) ;
#25097=COLOUR_RGB('Steel - Galvanized (Small)', 0.31764706, 0.68627451, 0.89019608) ;
ENDSEC;
END-ISO-10303-21;
